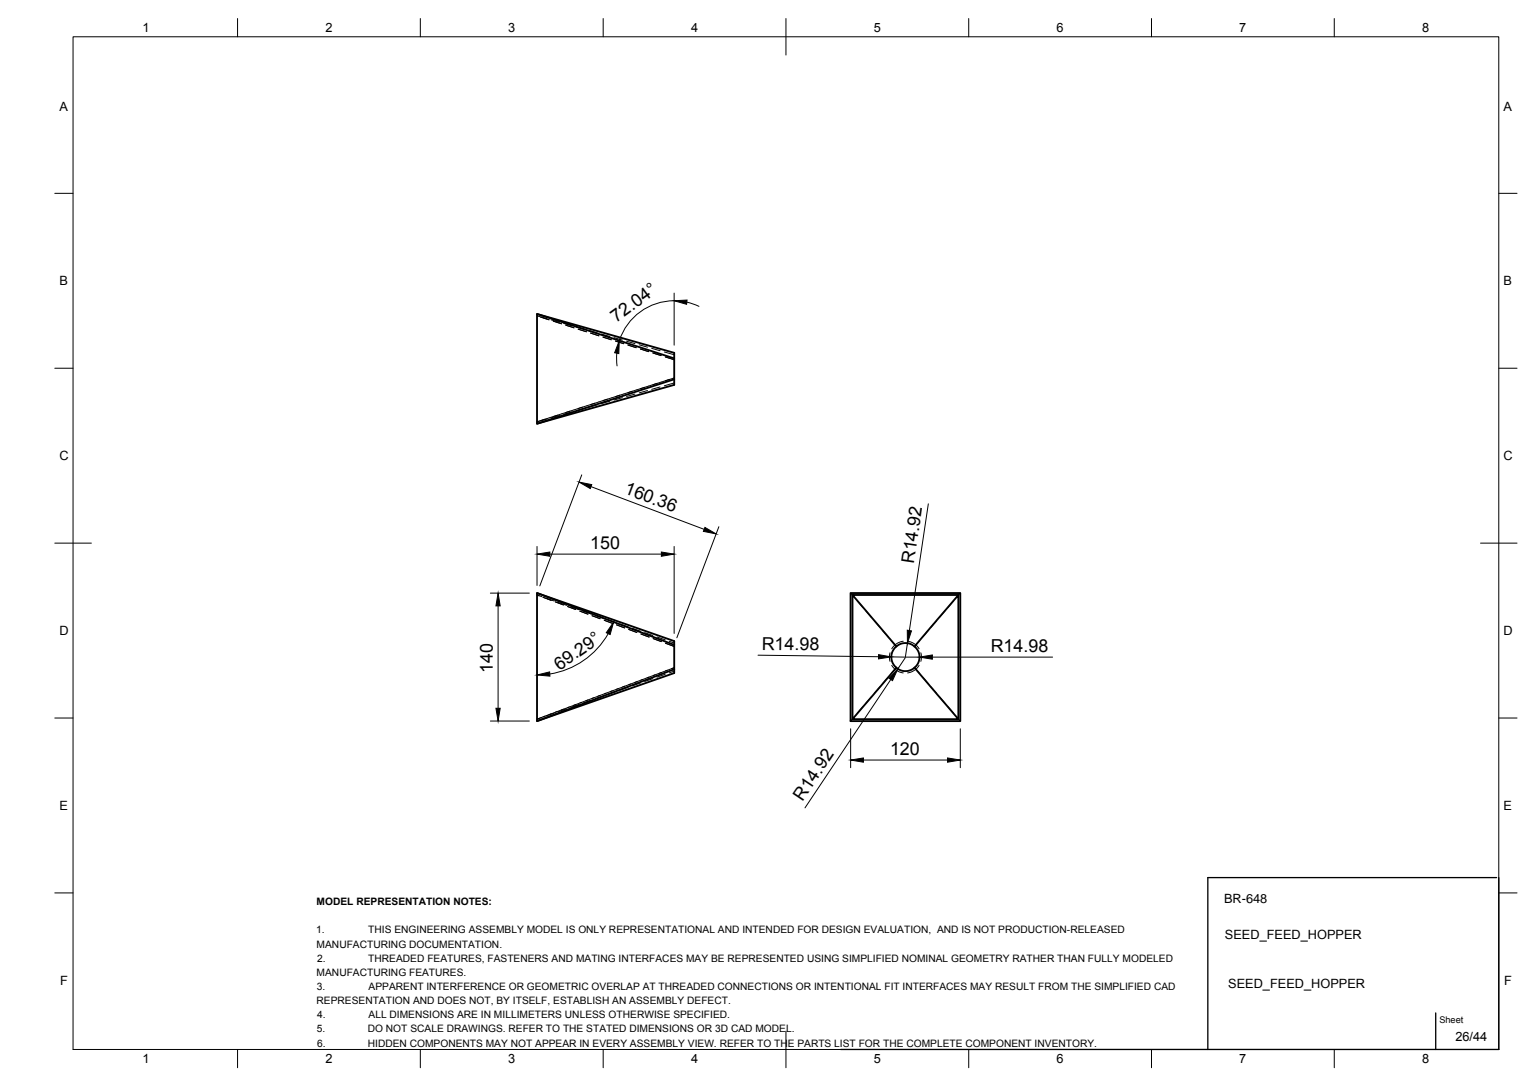
ISO-10303-21;
HEADER;
FILE_DESCRIPTION((''),'2;1');
FILE_NAME('SEED_FEED_HOPPER.step','2026-10-01T22:05:39-07:00',(''),(''),'','','');
FILE_SCHEMA (('AUTOMOTIVE_DESIGN { 1 0 10303 214 3 1 1 }'));
ENDSEC;
DATA;
#10=MECHANICAL_DESIGN_GEOMETRIC_PRESENTATION_REPRESENTATION('',(#624),#24628);
#13=B_SPLINE_SURFACE_WITH_KNOTS('',3,3,((#22362,#22363,#22364,#22365,#22366,
#22367,#22368),(#22369,#22370,#22371,#22372,#22373,#22374,#22375),(#22376,
#22377,#22378,#22379,#22380,#22381,#22382),(#22383,#22384,#22385,#22386,
#22387,#22388,#22389),(#22390,#22391,#22392,#22393,#22394,#22395,#22396),
(#22397,#22398,#22399,#22400,#22401,#22402,#22403)),.UNSPECIFIED.,.F.,.F.,
 .F.,(4,1,1,4),(4,1,1,1,4),(-0.0016506318429804,0.2850068720673,0.571664375977581,
1.001650631843),(0.00440207412461945,0.433637210821686,0.71979396861973,
0.862872347518753,1.00595072641777),.UNSPECIFIED.) ;
#14=B_SPLINE_SURFACE_WITH_KNOTS('',3,3,((#22475,#22476,#22477,#22478,#22479,
#22480,#22481),(#22482,#22483,#22484,#22485,#22486,#22487,#22488),(#22489,
#22490,#22491,#22492,#22493,#22494,#22495),(#22496,#22497,#22498,#22499,
#22500,#22501,#22502),(#22503,#22504,#22505,#22506,#22507,#22508,#22509),
(#22510,#22511,#22512,#22513,#22514,#22515,#22516),(#22517,#22518,#22519,
#22520,#22521,#22522,#22523)),.UNSPECIFIED.,.F.,.F.,.F.,(4,1,1,1,4),(4,
1,1,1,4),(-0.00135073644513769,0.285135398666339,0.428378466222077,0.714864601333554,
1.00135073644503),(0.00363062073752213,0.433196670488858,0.719574036989748,
0.862762720240194,1.00595140349064),.UNSPECIFIED.) ;
#15=B_SPLINE_SURFACE_WITH_KNOTS('',3,3,((#22568,#22569,#22570,#22571,#22572,
#22573),(#22574,#22575,#22576,#22577,#22578,#22579),(#22580,#22581,#22582,
#22583,#22584,#22585),(#22586,#22587,#22588,#22589,#22590,#22591),(#22592,
#22593,#22594,#22595,#22596,#22597),(#22598,#22599,#22600,#22601,#22602,
#22603)),.UNSPECIFIED.,.F.,.F.,.F.,(4,1,1,4),(4,1,1,4),(-0.00165063184293244,
0.28500687206736,0.571664375977652,1.00165063184309),(0.00440207412461947,
0.576715589720881,0.862872347519012,1.00595072641808),.UNSPECIFIED.) ;
#16=B_SPLINE_SURFACE_WITH_KNOTS('',3,3,((#22646,#22647,#22648,#22649,#22650,
#22651,#22652),(#22653,#22654,#22655,#22656,#22657,#22658,#22659),(#22660,
#22661,#22662,#22663,#22664,#22665,#22666),(#22667,#22668,#22669,#22670,
#22671,#22672,#22673),(#22674,#22675,#22676,#22677,#22678,#22679,#22680),
(#22681,#22682,#22683,#22684,#22685,#22686,#22687),(#22688,#22689,#22690,
#22691,#22692,#22693,#22694)),.UNSPECIFIED.,.F.,.F.,.F.,(4,1,1,1,4),(4,
1,1,1,4),(-0.00135073644515613,0.141892331110593,0.428378466222092,0.714864601333591,
1.00135073644509),(0.00363062073752213,0.433196670488988,0.719574036989965,
0.862762720240453,1.00595140349094),.UNSPECIFIED.) ;
#17=B_SPLINE_SURFACE_WITH_KNOTS('',3,3,((#22731,#22732,#22733,#22734),(#22735,
#22736,#22737,#22738),(#22739,#22740,#22741,#22742),(#22743,#22744,#22745,
#22746),(#22747,#22748,#22749,#22750),(#22751,#22752,#22753,#22754)),
 .UNSPECIFIED.,.F.,.F.,.F.,(4,1,1,4),(4,4),(0.,0.285714285714286,0.571428571428571,
1.),(0.,1.),.UNSPECIFIED.) ;
#18=B_SPLINE_SURFACE_WITH_KNOTS('',3,3,((#22757,#22758,#22759,#22760),(#22761,
#22762,#22763,#22764),(#22765,#22766,#22767,#22768),(#22769,#22770,#22771,
#22772),(#22773,#22774,#22775,#22776),(#22777,#22778,#22779,#22780),(#22781,
#22782,#22783,#22784)),.UNSPECIFIED.,.F.,.F.,.F.,(4,1,1,1,4),(4,4),(0.,
0.285714285714286,0.571428571428571,0.857142857142857,1.),(0.,1.),
 .UNSPECIFIED.) ;
#19=B_SPLINE_SURFACE_WITH_KNOTS('',3,3,((#22786,#22787,#22788,#22789),(#22790,
#22791,#22792,#22793),(#22794,#22795,#22796,#22797),(#22798,#22799,#22800,
#22801),(#22802,#22803,#22804,#22805),(#22806,#22807,#22808,#22809)),
 .UNSPECIFIED.,.F.,.F.,.F.,(4,1,1,4),(4,4),(0.,0.285714285714286,0.571428571428571,
1.),(0.,1.),.UNSPECIFIED.) ;
#20=B_SPLINE_SURFACE_WITH_KNOTS('',3,3,((#22811,#22812,#22813,#22814),(#22815,
#22816,#22817,#22818),(#22819,#22820,#22821,#22822),(#22823,#22824,#22825,
#22826),(#22827,#22828,#22829,#22830),(#22831,#22832,#22833,#22834),(#22835,
#22836,#22837,#22838)),.UNSPECIFIED.,.F.,.F.,.F.,(4,1,1,1,4),(4,4),(0.,
0.285714285714286,0.571428571428571,0.857142857142857,1.),(0.,1.),
 .UNSPECIFIED.) ;
#540=SHAPE_REPRESENTATION_RELATIONSHIP('SRR','None',#24813,#582) ;
#582=ADVANCED_BREP_SHAPE_REPRESENTATION('',(#663),#24603) ;
#624=STYLED_ITEM('',(#25038),#663) ;
#663=MANIFOLD_SOLID_BREP('SEED_FEED_HOPPER',#13166) ;
#871=FACE_BOUND('',#4402,.T.) ;
#872=FACE_BOUND('',#4404,.T.) ;
#964=B_SPLINE_CURVE_WITH_KNOTS('',3,(#22406,#22407,#22408,#22409,#22410,
#22411),.UNSPECIFIED.,.F.,.F.,(4,2,4),(0.306797486954004,6.07243999004955,
11.9854458646039),.UNSPECIFIED.) ;
#965=B_SPLINE_CURVE_WITH_KNOTS('',3,(#22413,#22414,#22415,#22416,#22417,
#22418,#22419,#22420,#22421,#22422,#22423,#22424,#22425,#22426,#22427,#22428),
 .UNSPECIFIED.,.F.,.F.,(4,3,3,3,3,4),(-22.7491660875703,-22.7326322777483,
-11.3663161388741,-8.43127796455208,-7.52321841795695,-0.0683548158626444),
 .UNSPECIFIED.) ;
#966=B_SPLINE_CURVE_WITH_KNOTS('',3,(#22430,#22431,#22432,#22433,#22434,
#22435,#22436),.UNSPECIFIED.,.F.,.F.,(4,3,4),(0.149401224909902,0.242876764795977,
0.248953560391612),.UNSPECIFIED.) ;
#967=B_SPLINE_CURVE_WITH_KNOTS('',3,(#22438,#22439,#22440,#22441,#22442,
#22443,#22444,#22445,#22446,#22447),.UNSPECIFIED.,.F.,.F.,(4,2,2,2,4),(0.0182113449411267,
0.579498375271715,1.16103870949885,1.68899220567266,2.20049000979166),
 .UNSPECIFIED.) ;
#968=B_SPLINE_CURVE_WITH_KNOTS('',3,(#22449,#22450,#22451,#22452,#22453,
#22454,#22455),.UNSPECIFIED.,.F.,.F.,(4,3,4),(-0.00607546474194351,0.,0.0934550397936403),
 .UNSPECIFIED.) ;
#969=B_SPLINE_CURVE_WITH_KNOTS('',3,(#22456,#22457,#22458,#22459,#22460,
#22461,#22462,#22463,#22464,#22465,#22466,#22467,#22468,#22469,#22470,#22471,
#22472,#22473,#22474),.UNSPECIFIED.,.F.,.F.,(4,3,3,3,3,3,4),(-8.32916619482315,
-6.19701983076071,-5.68275153370131,-5.33626613109357,-0.491091685615563,
0.,0.00607621245833095),.UNSPECIFIED.) ;
#970=B_SPLINE_CURVE_WITH_KNOTS('',3,(#22525,#22526,#22527,#22528,#22529,
#22530),.UNSPECIFIED.,.F.,.F.,(4,2,4),(0.330130434724689,7.1450073655251,
14.1316592404919),.UNSPECIFIED.) ;
#971=B_SPLINE_CURVE_WITH_KNOTS('',3,(#22532,#22533,#22534,#22535,#22536,
#22537,#22538,#22539,#22540,#22541,#22542,#22543,#22544,#22545,#22546,#22547),
 .UNSPECIFIED.,.F.,.F.,(4,3,3,3,3,4),(-0.00607619681590831,0.,4.17713740634383,
5.25576768694509,5.58948106622994,8.32915431888067),.UNSPECIFIED.) ;
#972=B_SPLINE_CURVE_WITH_KNOTS('',3,(#22549,#22550,#22551,#22552,#22553,
#22554,#22555),.UNSPECIFIED.,.F.,.F.,(4,3,4),(-0.093455064791989,0.,0.00607547210165982),
 .UNSPECIFIED.) ;
#973=B_SPLINE_CURVE_WITH_KNOTS('',3,(#22556,#22557,#22558,#22559,#22560,
#22561,#22562,#22563,#22564,#22565,#22566,#22567),.UNSPECIFIED.,.F.,.F.,
(4,2,2,2,2,4),(0.0230676064321383,0.582322749083777,1.16480388155931,1.75243736265584,
2.22755255780229,2.68204291945575),.UNSPECIFIED.) ;
#974=B_SPLINE_CURVE_WITH_KNOTS('',3,(#22605,#22606,#22607,#22608,#22609,
#22610),.UNSPECIFIED.,.F.,.F.,(4,2,4),(0.306797486954258,6.07243999011767,
11.9854458647428),.UNSPECIFIED.) ;
#975=B_SPLINE_CURVE_WITH_KNOTS('',3,(#22612,#22613,#22614,#22615,#22616,
#22617,#22618,#22619,#22620,#22621,#22622,#22623,#22624,#22625,#22626,#22627),
 .UNSPECIFIED.,.F.,.F.,(4,3,3,3,3,4),(-22.7491696598115,-22.732635833168,
-11.366317916584,-8.43127594084112,-7.52321777514952,-0.0683548158626444),
 .UNSPECIFIED.) ;
#976=B_SPLINE_CURVE_WITH_KNOTS('',3,(#22629,#22630,#22631,#22632,#22633,
#22634,#22635),.UNSPECIFIED.,.F.,.F.,(4,3,4),(0.149401210175699,0.242876791624169,
0.248953579588731),.UNSPECIFIED.) ;
#977=B_SPLINE_CURVE_WITH_KNOTS('',3,(#22636,#22637,#22638,#22639,#22640,
#22641,#22642,#22643,#22644,#22645),.UNSPECIFIED.,.F.,.F.,(4,2,2,2,4),(0.0182113449411156,
0.579498375271719,1.16103870949884,1.68899220567264,2.20049000979168),
 .UNSPECIFIED.) ;
#978=B_SPLINE_CURVE_WITH_KNOTS('',3,(#22695,#22696,#22697,#22698,#22699,
#22700),.UNSPECIFIED.,.F.,.F.,(4,2,4),(0.330130434724726,7.14500736553715,
14.1316592405166),.UNSPECIFIED.) ;
#979=B_SPLINE_CURVE_WITH_KNOTS('',3,(#22701,#22702,#22703,#22704,#22705,
#22706,#22707,#22708,#22709,#22710,#22711,#22712),.UNSPECIFIED.,.F.,.F.,
(4,2,2,2,2,4),(0.0230676064320783,0.582322749083774,1.1648038815593,1.75243736265581,
2.22755255780225,2.68204291945565),.UNSPECIFIED.) ;
#1442=LINE('',#22725,#2278) ;
#1443=LINE('',#22727,#2279) ;
#1444=LINE('',#22729,#2280) ;
#1445=LINE('',#22730,#2281) ;
#1446=LINE('',#22755,#2282) ;
#1447=LINE('',#22756,#2283) ;
#1448=LINE('',#22785,#2284) ;
#1449=LINE('',#22810,#2285) ;
#2278=VECTOR('',#18253,1.) ;
#2279=VECTOR('',#18254,1.) ;
#2280=VECTOR('',#18255,1.) ;
#2281=VECTOR('',#18256,1.) ;
#2282=VECTOR('',#18257,16.7569118395806) ;
#2283=VECTOR('',#18258,16.7569118395806) ;
#2284=VECTOR('',#18259,16.7569118395806) ;
#2285=VECTOR('',#18260,16.7569118395806) ;
#3445=FACE_OUTER_BOUND('',#4397,.T.) ;
#3446=FACE_OUTER_BOUND('',#4398,.T.) ;
#3447=FACE_OUTER_BOUND('',#4399,.T.) ;
#3448=FACE_OUTER_BOUND('',#4400,.T.) ;
#3449=FACE_OUTER_BOUND('',#4401,.T.) ;
#3450=FACE_OUTER_BOUND('',#4403,.T.) ;
#3451=FACE_OUTER_BOUND('',#4405,.T.) ;
#3452=FACE_OUTER_BOUND('',#4406,.T.) ;
#3453=FACE_OUTER_BOUND('',#4407,.T.) ;
#3454=FACE_OUTER_BOUND('',#4408,.T.) ;
#4397=EDGE_LOOP('',(#10729,#10730,#10731,#10732,#10733,#10734)) ;
#4398=EDGE_LOOP('',(#10735,#10736,#10737,#10738,#10739,#10740)) ;
#4399=EDGE_LOOP('',(#10741,#10742,#10743,#10744,#10745,#10746)) ;
#4400=EDGE_LOOP('',(#10747,#10748,#10749,#10750,#10751,#10752)) ;
#4401=EDGE_LOOP('',(#10753,#10754,#10755,#10756)) ;
#4402=EDGE_LOOP('',(#10757,#10758,#10759,#10760)) ;
#4403=EDGE_LOOP('',(#10761,#10762,#10763,#10764)) ;
#4404=EDGE_LOOP('',(#10765,#10766,#10767,#10768)) ;
#4405=EDGE_LOOP('',(#10769,#10770,#10771,#10772)) ;
#4406=EDGE_LOOP('',(#10773,#10774,#10775,#10776)) ;
#4407=EDGE_LOOP('',(#10777,#10778,#10779,#10780)) ;
#4408=EDGE_LOOP('',(#10781,#10782,#10783,#10784)) ;
#5342=CIRCLE('',#14858,1.75) ;
#5343=CIRCLE('',#14859,1.75) ;
#5344=CIRCLE('',#14860,1.75) ;
#5345=CIRCLE('',#14861,1.75) ;
#6312=VERTEX_POINT('',#22404) ;
#6313=VERTEX_POINT('',#22405) ;
#6314=VERTEX_POINT('',#22412) ;
#6315=VERTEX_POINT('',#22429) ;
#6316=VERTEX_POINT('',#22437) ;
#6317=VERTEX_POINT('',#22448) ;
#6318=VERTEX_POINT('',#22524) ;
#6319=VERTEX_POINT('',#22531) ;
#6320=VERTEX_POINT('',#22548) ;
#6321=VERTEX_POINT('',#22604) ;
#6322=VERTEX_POINT('',#22611) ;
#6323=VERTEX_POINT('',#22628) ;
#6324=VERTEX_POINT('',#22714) ;
#6325=VERTEX_POINT('',#22715) ;
#6326=VERTEX_POINT('',#22717) ;
#6327=VERTEX_POINT('',#22719) ;
#6328=VERTEX_POINT('',#22723) ;
#6329=VERTEX_POINT('',#22724) ;
#6330=VERTEX_POINT('',#22726) ;
#6331=VERTEX_POINT('',#22728) ;
#7854=EDGE_CURVE('',#6312,#6313,#964,.T.) ;
#7855=EDGE_CURVE('',#6312,#6314,#965,.F.) ;
#7856=EDGE_CURVE('',#6314,#6315,#966,.F.) ;
#7857=EDGE_CURVE('',#6316,#6315,#967,.T.) ;
#7858=EDGE_CURVE('',#6317,#6316,#968,.T.) ;
#7859=EDGE_CURVE('',#6313,#6317,#969,.T.) ;
#7860=EDGE_CURVE('',#6318,#6312,#970,.T.) ;
#7861=EDGE_CURVE('',#6318,#6319,#971,.F.) ;
#7862=EDGE_CURVE('',#6319,#6320,#972,.F.) ;
#7863=EDGE_CURVE('',#6315,#6320,#973,.T.) ;
#7864=EDGE_CURVE('',#6321,#6318,#974,.T.) ;
#7865=EDGE_CURVE('',#6321,#6322,#975,.F.) ;
#7866=EDGE_CURVE('',#6322,#6323,#976,.F.) ;
#7867=EDGE_CURVE('',#6320,#6323,#977,.T.) ;
#7868=EDGE_CURVE('',#6313,#6321,#978,.T.) ;
#7869=EDGE_CURVE('',#6323,#6316,#979,.T.) ;
#7870=EDGE_CURVE('',#6324,#6325,#5342,.T.) ;
#7871=EDGE_CURVE('',#6326,#6324,#5343,.T.) ;
#7872=EDGE_CURVE('',#6327,#6326,#5344,.T.) ;
#7873=EDGE_CURVE('',#6325,#6327,#5345,.T.) ;
#7874=EDGE_CURVE('',#6328,#6329,#1442,.T.) ;
#7875=EDGE_CURVE('',#6329,#6330,#1443,.T.) ;
#7876=EDGE_CURVE('',#6330,#6331,#1444,.T.) ;
#7877=EDGE_CURVE('',#6331,#6328,#1445,.T.) ;
#7878=EDGE_CURVE('',#6328,#6324,#1446,.T.) ;
#7879=EDGE_CURVE('',#6329,#6325,#1447,.T.) ;
#7880=EDGE_CURVE('',#6330,#6327,#1448,.T.) ;
#7881=EDGE_CURVE('',#6331,#6326,#1449,.T.) ;
#10729=ORIENTED_EDGE('',*,*,#7854,.F.) ;
#10730=ORIENTED_EDGE('',*,*,#7855,.T.) ;
#10731=ORIENTED_EDGE('',*,*,#7856,.T.) ;
#10732=ORIENTED_EDGE('',*,*,#7857,.F.) ;
#10733=ORIENTED_EDGE('',*,*,#7858,.F.) ;
#10734=ORIENTED_EDGE('',*,*,#7859,.F.) ;
#10735=ORIENTED_EDGE('',*,*,#7860,.F.) ;
#10736=ORIENTED_EDGE('',*,*,#7861,.T.) ;
#10737=ORIENTED_EDGE('',*,*,#7862,.T.) ;
#10738=ORIENTED_EDGE('',*,*,#7863,.F.) ;
#10739=ORIENTED_EDGE('',*,*,#7856,.F.) ;
#10740=ORIENTED_EDGE('',*,*,#7855,.F.) ;
#10741=ORIENTED_EDGE('',*,*,#7864,.F.) ;
#10742=ORIENTED_EDGE('',*,*,#7865,.T.) ;
#10743=ORIENTED_EDGE('',*,*,#7866,.T.) ;
#10744=ORIENTED_EDGE('',*,*,#7867,.F.) ;
#10745=ORIENTED_EDGE('',*,*,#7862,.F.) ;
#10746=ORIENTED_EDGE('',*,*,#7861,.F.) ;
#10747=ORIENTED_EDGE('',*,*,#7868,.F.) ;
#10748=ORIENTED_EDGE('',*,*,#7859,.T.) ;
#10749=ORIENTED_EDGE('',*,*,#7858,.T.) ;
#10750=ORIENTED_EDGE('',*,*,#7869,.F.) ;
#10751=ORIENTED_EDGE('',*,*,#7866,.F.) ;
#10752=ORIENTED_EDGE('',*,*,#7865,.F.) ;
#10753=ORIENTED_EDGE('',*,*,#7870,.F.) ;
#10754=ORIENTED_EDGE('',*,*,#7871,.F.) ;
#10755=ORIENTED_EDGE('',*,*,#7872,.F.) ;
#10756=ORIENTED_EDGE('',*,*,#7873,.F.) ;
#10757=ORIENTED_EDGE('',*,*,#7857,.T.) ;
#10758=ORIENTED_EDGE('',*,*,#7863,.T.) ;
#10759=ORIENTED_EDGE('',*,*,#7867,.T.) ;
#10760=ORIENTED_EDGE('',*,*,#7869,.T.) ;
#10761=ORIENTED_EDGE('',*,*,#7874,.T.) ;
#10762=ORIENTED_EDGE('',*,*,#7875,.T.) ;
#10763=ORIENTED_EDGE('',*,*,#7876,.T.) ;
#10764=ORIENTED_EDGE('',*,*,#7877,.T.) ;
#10765=ORIENTED_EDGE('',*,*,#7854,.T.) ;
#10766=ORIENTED_EDGE('',*,*,#7868,.T.) ;
#10767=ORIENTED_EDGE('',*,*,#7864,.T.) ;
#10768=ORIENTED_EDGE('',*,*,#7860,.T.) ;
#10769=ORIENTED_EDGE('',*,*,#7874,.F.) ;
#10770=ORIENTED_EDGE('',*,*,#7878,.T.) ;
#10771=ORIENTED_EDGE('',*,*,#7870,.T.) ;
#10772=ORIENTED_EDGE('',*,*,#7879,.F.) ;
#10773=ORIENTED_EDGE('',*,*,#7875,.F.) ;
#10774=ORIENTED_EDGE('',*,*,#7879,.T.) ;
#10775=ORIENTED_EDGE('',*,*,#7873,.T.) ;
#10776=ORIENTED_EDGE('',*,*,#7880,.F.) ;
#10777=ORIENTED_EDGE('',*,*,#7876,.F.) ;
#10778=ORIENTED_EDGE('',*,*,#7880,.T.) ;
#10779=ORIENTED_EDGE('',*,*,#7872,.T.) ;
#10780=ORIENTED_EDGE('',*,*,#7881,.F.) ;
#10781=ORIENTED_EDGE('',*,*,#7877,.F.) ;
#10782=ORIENTED_EDGE('',*,*,#7881,.T.) ;
#10783=ORIENTED_EDGE('',*,*,#7871,.T.) ;
#10784=ORIENTED_EDGE('',*,*,#7878,.F.) ;
#12164=PLANE('',#14857) ;
#12165=PLANE('',#14862) ;
#12840=ADVANCED_FACE('',(#3445),#13,.T.) ;
#12841=ADVANCED_FACE('',(#3446),#14,.T.) ;
#12842=ADVANCED_FACE('',(#3447),#15,.T.) ;
#12843=ADVANCED_FACE('',(#3448),#16,.T.) ;
#12844=ADVANCED_FACE('',(#3449,#871),#12164,.F.) ;
#12845=ADVANCED_FACE('',(#3450,#872),#12165,.T.) ;
#12846=ADVANCED_FACE('',(#3451),#17,.F.) ;
#12847=ADVANCED_FACE('',(#3452),#18,.F.) ;
#12848=ADVANCED_FACE('',(#3453),#19,.F.) ;
#12849=ADVANCED_FACE('',(#3454),#20,.F.) ;
#13166=CLOSED_SHELL('',(#12840,#12841,#12842,#12843,#12844,#12845,#12846,
#12847,#12848,#12849)) ;
#14856=AXIS2_PLACEMENT_3D('',#22361,#18239,#18240) ;
#14857=AXIS2_PLACEMENT_3D('',#22713,#18241,#18242) ;
#14858=AXIS2_PLACEMENT_3D('',#22716,#18243,#18244) ;
#14859=AXIS2_PLACEMENT_3D('',#22718,#18245,#18246) ;
#14860=AXIS2_PLACEMENT_3D('',#22720,#18247,#18248) ;
#14861=AXIS2_PLACEMENT_3D('',#22721,#18249,#18250) ;
#14862=AXIS2_PLACEMENT_3D('',#22722,#18251,#18252) ;
#18239=DIRECTION('axis',(0.,0.,1.)) ;
#18240=DIRECTION('refdir',(1.,0.,0.)) ;
#18241=DIRECTION('center_axis',(0.,0.,1.)) ;
#18242=DIRECTION('ref_axis',(1.,0.,0.)) ;
#18243=DIRECTION('center_axis',(0.,0.,1.)) ;
#18244=DIRECTION('ref_axis',(1.,0.,0.)) ;
#18245=DIRECTION('center_axis',(0.,0.,1.)) ;
#18246=DIRECTION('ref_axis',(1.,0.,0.)) ;
#18247=DIRECTION('center_axis',(0.,0.,1.)) ;
#18248=DIRECTION('ref_axis',(1.,0.,0.)) ;
#18249=DIRECTION('center_axis',(0.,0.,1.)) ;
#18250=DIRECTION('ref_axis',(1.,0.,0.)) ;
#18251=DIRECTION('center_axis',(0.,0.,1.)) ;
#18252=DIRECTION('ref_axis',(1.,0.,0.)) ;
#18253=DIRECTION('',(0.,-1.,0.)) ;
#18254=DIRECTION('',(1.,0.,0.)) ;
#18255=DIRECTION('',(0.,1.,0.)) ;
#18256=DIRECTION('',(-1.,-6.34413156928661E-17,0.)) ;
#18257=DIRECTION('',(0.338445472540165,-0.290096119320142,-0.895153005732796)) ;
#18258=DIRECTION('',(0.338445472540165,0.290096119320142,-0.895153005732796)) ;
#18259=DIRECTION('',(-0.338445472540165,0.290096119320142,-0.895153005732796)) ;
#18260=DIRECTION('',(-0.338445472540165,-0.290096119320142,-0.895153005732796)) ;
#22361=CARTESIAN_POINT('',(0.,0.,0.)) ;
#22362=CARTESIAN_POINT('Ctrl Pts',(-29.7879704997762,4.1982235964065,15.004760387006)) ;
#22363=CARTESIAN_POINT('Ctrl Pts',(-28.9765416158345,3.49667700708559,12.8596184051575)) ;
#22364=CARTESIAN_POINT('Ctrl Pts',(-27.6245525523466,2.32566824542574,9.28480711044218)) ;
#22365=CARTESIAN_POINT('Ctrl Pts',(-26.005233549839,0.90734538201738,4.99813706529367)) ;
#22366=CARTESIAN_POINT('Ctrl Pts',(-24.9352460971343,-0.0565633455803164,
2.14271187262585)) ;
#22367=CARTESIAN_POINT('Ctrl Pts',(-24.4110437339872,-0.552959968693851,
0.715613732723115)) ;
#22368=CARTESIAN_POINT('Ctrl Pts',(-24.1589049321087,-0.806397566452131,
-5.70268832156273E-10)) ;
#22369=CARTESIAN_POINT('Ctrl Pts',(-29.7880085856475,3.05586778828661,15.0030622151785)) ;
#22370=CARTESIAN_POINT('Ctrl Pts',(-28.9985961339778,2.49325092521034,12.8575620409374)) ;
#22371=CARTESIAN_POINT('Ctrl Pts',(-27.6830843893262,1.55403581881225,9.28200460526821)) ;
#22372=CARTESIAN_POINT('Ctrl Pts',(-26.1062403134519,0.416417293310764,
4.99328651815293)) ;
#22373=CARTESIAN_POINT('Ctrl Pts',(-25.0612351613324,-0.357449889914694,
2.13576141937932)) ;
#22374=CARTESIAN_POINT('Ctrl Pts',(-24.5450981755029,-0.75720095086868,
0.707828841054705)) ;
#22375=CARTESIAN_POINT('Ctrl Pts',(-24.2953334946171,-0.964113147540073,
-0.00706604193771441)) ;
#22376=CARTESIAN_POINT('Ctrl Pts',(-29.7880984019284,0.77088432617787,15.0004371510981)) ;
#22377=CARTESIAN_POINT('Ctrl Pts',(-29.0320656779143,0.477248554069186,
12.854352481685)) ;
#22378=CARTESIAN_POINT('Ctrl Pts',(-27.7718140786327,-0.0129653268429286,
9.2776079223855)) ;
#22379=CARTESIAN_POINT('Ctrl Pts',(-26.2598801085757,-0.606556867865899,
4.9857552974963)) ;
#22380=CARTESIAN_POINT('Ctrl Pts',(-25.252746996273,-1.01128931246026,2.12475519883151)) ;
#22381=CARTESIAN_POINT('Ctrl Pts',(-24.7498599068977,-1.22062620685322,
0.694492730733407)) ;
#22382=CARTESIAN_POINT('Ctrl Pts',(-24.5000082407848,-1.33280874531094,
-0.0206610680077742)) ;
#22383=CARTESIAN_POINT('Ctrl Pts',(-29.7881434031396,-3.22828201380981,
14.9994444092913)) ;
#22384=CARTESIAN_POINT('Ctrl Pts',(-29.0444129979685,-3.06557811875762,
12.8531317839584)) ;
#22385=CARTESIAN_POINT('Ctrl Pts',(-27.8048257006081,-2.79391277080305,
9.27588292843548)) ;
#22386=CARTESIAN_POINT('Ctrl Pts',(-26.317044506741,-2.46505212911362,4.98280140110366)) ;
#22387=CARTESIAN_POINT('Ctrl Pts',(-25.3239448603091,-2.24067401478496,
2.12040334815057)) ;
#22388=CARTESIAN_POINT('Ctrl Pts',(-24.8262703953289,-2.12469662243215,
0.688894444476874)) ;
#22389=CARTESIAN_POINT('Ctrl Pts',(-24.5752760211477,-2.06194576114233,
-0.0267624859759424)) ;
#22390=CARTESIAN_POINT('Ctrl Pts',(-29.7880276285832,-6.08468988422692,
15.0022131292648)) ;
#22391=CARTESIAN_POINT('Ctrl Pts',(-29.0097274305354,-5.59160872404636,
12.8565299181811)) ;
#22392=CARTESIAN_POINT('Ctrl Pts',(-27.7122818351144,-4.76817410676846,
9.28063964648335)) ;
#22393=CARTESIAN_POINT('Ctrl Pts',(-26.1568276984181,-3.77112949936236,
4.99094264430357)) ;
#22394=CARTESIAN_POINT('Ctrl Pts',(-25.1243483646472,-3.09226178271257,
2.13236773367943)) ;
#22395=CARTESIAN_POINT('Ctrl Pts',(-24.6123236175051,-2.74112531762835,
0.704011231405586)) ;
#22396=CARTESIAN_POINT('Ctrl Pts',(-24.3635477758713,-2.557029061916,-0.0105990626214356)) ;
#22397=CARTESIAN_POINT('Ctrl Pts',(-29.7879704997762,-7.79822359640676,
15.004760387006)) ;
#22398=CARTESIAN_POINT('Ctrl Pts',(-28.9765416158345,-7.09667700708582,
12.8596184051575)) ;
#22399=CARTESIAN_POINT('Ctrl Pts',(-27.6245525523466,-5.92566824542591,
9.28480711044218)) ;
#22400=CARTESIAN_POINT('Ctrl Pts',(-26.0052335498389,-4.50734538201749,
4.99813706529367)) ;
#22401=CARTESIAN_POINT('Ctrl Pts',(-24.9352460971343,-3.54343665441975,
2.14271187262586)) ;
#22402=CARTESIAN_POINT('Ctrl Pts',(-24.4110437339872,-3.0470400313062,0.715613732723117)) ;
#22403=CARTESIAN_POINT('Ctrl Pts',(-24.1589049321087,-2.79360243354791,
-5.70267222332888E-10)) ;
#22404=CARTESIAN_POINT('',(-29.7862997944388,-7.58988663107372,15.)) ;
#22405=CARTESIAN_POINT('',(-29.7862997944388,3.98988663107372,15.)) ;
#22406=CARTESIAN_POINT('Ctrl Pts',(-29.7862997944388,-7.58988663107372,
15.)) ;
#22407=CARTESIAN_POINT('Ctrl Pts',(-29.7874854452745,-5.67140621570733,
15.)) ;
#22408=CARTESIAN_POINT('Ctrl Pts',(-29.7880884026998,-3.78346330304678,
15.)) ;
#22409=CARTESIAN_POINT('Ctrl Pts',(-29.7881190038692,0.0862220953979725,
15.)) ;
#22410=CARTESIAN_POINT('Ctrl Pts',(-29.7875160987196,2.02180642423597,15.)) ;
#22411=CARTESIAN_POINT('Ctrl Pts',(-29.7862997944388,3.98988663107372,15.)) ;
#22412=CARTESIAN_POINT('',(-24.1927688881933,-2.82237333273713,0.0891518022986763)) ;
#22413=CARTESIAN_POINT('Ctrl Pts',(-24.1927688881933,-2.82237333273713,
0.0891518022986763)) ;
#22414=CARTESIAN_POINT('Ctrl Pts',(-24.1934570101164,-2.82295781734209,
0.0909648418835227)) ;
#22415=CARTESIAN_POINT('Ctrl Pts',(-24.1941451106354,-2.82354227530196,
0.092777911525871)) ;
#22416=CARTESIAN_POINT('Ctrl Pts',(-24.1948331817638,-2.82412669991032,
0.094590989728832)) ;
#22417=CARTESIAN_POINT('Ctrl Pts',(-24.6678538621346,-3.22589464870741,
1.34100789310195)) ;
#22418=CARTESIAN_POINT('Ctrl Pts',(-25.0587313958119,-3.55537106707809,
2.39676629444992)) ;
#22419=CARTESIAN_POINT('Ctrl Pts',(-26.0013963074572,-4.35779250443395,
4.91745743939535)) ;
#22420=CARTESIAN_POINT('Ctrl Pts',(-26.2448135648579,-4.56499574616668,
5.56835652100608)) ;
#22421=CARTESIAN_POINT('Ctrl Pts',(-26.5249696032859,-4.803694805458,6.31696827513027)) ;
#22422=CARTESIAN_POINT('Ctrl Pts',(-26.852785444491,-5.0833030095669,7.19178833495937)) ;
#22423=CARTESIAN_POINT('Ctrl Pts',(-26.9542070569034,-5.16980985682658,
7.46244536212537)) ;
#22424=CARTESIAN_POINT('Ctrl Pts',(-27.0601952624917,-5.26023714996938,
7.74519169930263)) ;
#22425=CARTESIAN_POINT('Ctrl Pts',(-27.1656849213349,-5.35026234294172,
8.02651094121919)) ;
#22426=CARTESIAN_POINT('Ctrl Pts',(-28.0317195564602,-6.0893389121793,10.3360473422142)) ;
#22427=CARTESIAN_POINT('Ctrl Pts',(-28.9467094713777,-6.87166395755108,
12.769529848754)) ;
#22428=CARTESIAN_POINT('Ctrl Pts',(-29.7862997944388,-7.58988663107372,
15.)) ;
#22429=CARTESIAN_POINT('',(-24.1589049319639,-2.79360243342489,-4.75519821435677E-10)) ;
#22430=CARTESIAN_POINT('Ctrl Pts',(-24.1589049321088,-2.79360243354777,
-5.70273040595426E-10)) ;
#22431=CARTESIAN_POINT('Ctrl Pts',(-24.1695174648536,-2.80262121435912,
0.0279159200689838)) ;
#22432=CARTESIAN_POINT('Ctrl Pts',(-24.1801188171535,-2.81162839675808,
0.0558294517448662)) ;
#22433=CARTESIAN_POINT('Ctrl Pts',(-24.1907006565412,-2.82061729735981,
0.083715933657329)) ;
#22434=CARTESIAN_POINT('Ctrl Pts',(-24.1913885763442,-2.82120166105167,
0.0855288191530417)) ;
#22435=CARTESIAN_POINT('Ctrl Pts',(-24.1920764667909,-2.82178599256751,
0.0873417302858431)) ;
#22436=CARTESIAN_POINT('Ctrl Pts',(-24.1927643256631,-2.8223702901168,0.0891546605139208)) ;
#22437=CARTESIAN_POINT('',(-24.1589049319644,-0.806397566574673,-4.7482698675716E-10)) ;
#22438=CARTESIAN_POINT('Ctrl Pts',(-24.1589049323255,-0.8063975662679,1.09620886621735E-16)) ;
#22439=CARTESIAN_POINT('Ctrl Pts',(-24.283597624207,-0.945716532508702,
1.09623628239148E-16)) ;
#22440=CARTESIAN_POINT('Ctrl Pts',(-24.3808054594196,-1.10713716355173,
-1.18390020009684E-12)) ;
#22441=CARTESIAN_POINT('Ctrl Pts',(-24.512802414918,-1.46434976621459,-1.18390020009684E-12)) ;
#22442=CARTESIAN_POINT('Ctrl Pts',(-24.5438655539448,-1.6575893537085,-1.38777878078145E-15)) ;
#22443=CARTESIAN_POINT('Ctrl Pts',(-24.5311976151215,-2.02703780425878,
-1.38777878078145E-15)) ;
#22444=CARTESIAN_POINT('Ctrl Pts',(-24.4941869311108,-2.20048822446343,
1.4585554986013E-14)) ;
#22445=CARTESIAN_POINT('Ctrl Pts',(-24.3634307218009,-2.52123101046768,
1.4585554986013E-14)) ;
#22446=CARTESIAN_POINT('Ctrl Pts',(-24.2725344551939,-2.66664433040153,
3.20484281317344E-16)) ;
#22447=CARTESIAN_POINT('Ctrl Pts',(-24.1589049323255,-2.79360243373209,
3.20484666411866E-16)) ;
#22448=CARTESIAN_POINT('',(-24.1927688881933,-0.777626667262871,0.0891518022986696)) ;
#22449=CARTESIAN_POINT('Ctrl Pts',(-24.1927640983708,-0.777630284368101,
0.0891545456106432)) ;
#22450=CARTESIAN_POINT('Ctrl Pts',(-24.1920762479986,-0.778214559997417,
0.0873416191464197)) ;
#22451=CARTESIAN_POINT('Ctrl Pts',(-24.1913883666309,-0.778798869477654,
0.0855287137798584)) ;
#22452=CARTESIAN_POINT('Ctrl Pts',(-24.1907004548719,-0.779383212398548,
0.0837158318083245)) ;
#22453=CARTESIAN_POINT('Ctrl Pts',(-24.1801187424362,-0.788371790761656,
0.0558294125816257)) ;
#22454=CARTESIAN_POINT('Ctrl Pts',(-24.1695174641247,-0.797378786260146,
0.0279159181518874)) ;
#22455=CARTESIAN_POINT('Ctrl Pts',(-24.158904932109,-0.806397566451893,
-5.69441659411157E-10)) ;
#22456=CARTESIAN_POINT('Ctrl Pts',(-29.7862997944388,3.98988663107372,15.)) ;
#22457=CARTESIAN_POINT('Ctrl Pts',(-29.1328907328544,3.43093163811475,13.2641422031832)) ;
#22458=CARTESIAN_POINT('Ctrl Pts',(-28.4338012516642,2.8331537658536,11.4053304313931)) ;
#22459=CARTESIAN_POINT('Ctrl Pts',(-27.7476813820024,2.24714826965254,9.5776689963089)) ;
#22460=CARTESIAN_POINT('Ctrl Pts',(-27.5821910090633,2.10580522975702,9.13684169211246)) ;
#22461=CARTESIAN_POINT('Ctrl Pts',(-27.4174547163538,1.96514782273,8.69782652065271)) ;
#22462=CARTESIAN_POINT('Ctrl Pts',(-27.2542924969021,1.82588555176052,8.26278713091792)) ;
#22463=CARTESIAN_POINT('Ctrl Pts',(-27.144362859745,1.73205837186077,7.96968176361375)) ;
#22464=CARTESIAN_POINT('Ctrl Pts',(-27.0345809892665,1.63838104542639,7.67686898630538)) ;
#22465=CARTESIAN_POINT('Ctrl Pts',(-26.926973332117,1.54658537416295,7.38975189096568)) ;
#22466=CARTESIAN_POINT('Ctrl Pts',(-25.4222119002236,0.262935219600215,
3.37477058806011)) ;
#22467=CARTESIAN_POINT('Ctrl Pts',(-24.8950276354157,-0.182007944164745,
1.94978881746105)) ;
#22468=CARTESIAN_POINT('Ctrl Pts',(-24.3591765397677,-0.636412221527215,
0.52907137988932)) ;
#22469=CARTESIAN_POINT('Ctrl Pts',(-24.304864353331,-0.682469213908392,
0.385071916288646)) ;
#22470=CARTESIAN_POINT('Ctrl Pts',(-24.2504445757749,-0.728638841618619,
0.241127884134561)) ;
#22471=CARTESIAN_POINT('Ctrl Pts',(-24.1948331817649,-0.775873300087209,
0.0945909897337519)) ;
#22472=CARTESIAN_POINT('Ctrl Pts',(-24.1941451093438,-0.776457725793072,
0.0927779081250757)) ;
#22473=CARTESIAN_POINT('Ctrl Pts',(-24.1934570114089,-0.777042181560007,
0.0909648452891593)) ;
#22474=CARTESIAN_POINT('Ctrl Pts',(-24.1927688881933,-0.777626667262871,
0.0891518022986696)) ;
#22475=CARTESIAN_POINT('Ctrl Pts',(-29.9981473192967,-7.59210557221634,
15.0072731137197)) ;
#22476=CARTESIAN_POINT('Ctrl Pts',(-29.1792583701285,-6.89610811582497,
12.86098396712)) ;
#22477=CARTESIAN_POINT('Ctrl Pts',(-27.8122956599382,-5.73660744609276,
9.28448922209497)) ;
#22478=CARTESIAN_POINT('Ctrl Pts',(-26.155155413787,-4.35020365083683,4.99743947373446)) ;
#22479=CARTESIAN_POINT('Ctrl Pts',(-25.0283996405944,-3.44029824352441,
2.14308849921247)) ;
#22480=CARTESIAN_POINT('Ctrl Pts',(-24.4500092405164,-3.00195022998226,
0.716220735767208)) ;
#22481=CARTESIAN_POINT('Ctrl Pts',(-24.1589049321088,-2.79360243354776,
-5.70272704059072E-10)) ;
#22482=CARTESIAN_POINT('Ctrl Pts',(-28.6654023870952,-7.59208088863895,
15.0047443273315)) ;
#22483=CARTESIAN_POINT('Ctrl Pts',(-28.0118306429454,-6.92739322509109,
12.8579428468339)) ;
#22484=CARTESIAN_POINT('Ctrl Pts',(-26.9205390890661,-5.81959198653294,
9.28039690179885)) ;
#22485=CARTESIAN_POINT('Ctrl Pts',(-25.5975062439661,-4.49340440306587,
4.99035344644854)) ;
#22486=CARTESIAN_POINT('Ctrl Pts',(-24.696887404406,-3.61843630935476,2.13290843001981)) ;
#22487=CARTESIAN_POINT('Ctrl Pts',(-24.231863933635,-3.19121227129626,0.705454724400515)) ;
#22488=CARTESIAN_POINT('Ctrl Pts',(-23.9940039875064,-2.98789208895153,
-0.00956374451382109)) ;
#22489=CARTESIAN_POINT('Ctrl Pts',(-26.6659920777596,-7.59211093203314,
15.0017046656488)) ;
#22490=CARTESIAN_POINT('Ctrl Pts',(-26.2487210328116,-6.96393546602423,
12.8542436051414)) ;
#22491=CARTESIAN_POINT('Ctrl Pts',(-25.551936157679,-5.91719526611694,9.27528884741571)) ;
#22492=CARTESIAN_POINT('Ctrl Pts',(-24.7073383684488,-4.66179365816894,
4.9815562676005)) ;
#22493=CARTESIAN_POINT('Ctrl Pts',(-24.131376536521,-3.82821717034421,2.12007028295518)) ;
#22494=CARTESIAN_POINT('Ctrl Pts',(-23.8331919862405,-3.4144691374418,0.689960097960527)) ;
#22495=CARTESIAN_POINT('Ctrl Pts',(-23.6762514799622,-3.21253192150677,
-0.0250972881037275)) ;
#22496=CARTESIAN_POINT('Ctrl Pts',(-23.3332927479438,-7.5921558493803,14.9995815283504)) ;
#22497=CARTESIAN_POINT('Ctrl Pts',(-23.2961810253174,-6.98936415220679,
12.8516417322129)) ;
#22498=CARTESIAN_POINT('Ctrl Pts',(-23.2341794813628,-5.98449411694383,
9.27170531871678)) ;
#22499=CARTESIAN_POINT('Ctrl Pts',(-23.1590806809098,-4.7786211064264,4.975481034806)) ;
#22500=CARTESIAN_POINT('Ctrl Pts',(-23.1077088424374,-3.97369033142903,
2.11102719571202)) ;
#22501=CARTESIAN_POINT('Ctrl Pts',(-23.0810207228591,-3.57040548608313,
0.678584002796474)) ;
#22502=CARTESIAN_POINT('Ctrl Pts',(-23.0663319046393,-3.36714380447418,
-0.037695190406408)) ;
#22503=CARTESIAN_POINT('Ctrl Pts',(-20.0004784533517,-7.59212538979759,
15.0006756318296)) ;
#22504=CARTESIAN_POINT('Ctrl Pts',(-20.3389974659838,-6.97635407369755,
12.8529859672692)) ;
#22505=CARTESIAN_POINT('Ctrl Pts',(-20.904309853669,-5.95003859913919,9.27357788116746)) ;
#22506=CARTESIAN_POINT('Ctrl Pts',(-21.589449075084,-4.71871053547002,4.97864159456366)) ;
#22507=CARTESIAN_POINT('Ctrl Pts',(-22.0572141827788,-3.89911706770722,
2.11576153158121)) ;
#22508=CARTESIAN_POINT('Ctrl Pts',(-22.2997449599209,-3.49018725280383,
0.68467274594701)) ;
#22509=CARTESIAN_POINT('Ctrl Pts',(-22.4296586836676,-3.28819168978624,
-0.0306758267980919)) ;
#22510=CARTESIAN_POINT('Ctrl Pts',(-17.3345976129064,-7.59208088863895,
15.0047443273315)) ;
#22511=CARTESIAN_POINT('Ctrl Pts',(-17.9881563810077,-6.92728037248107,
12.8579470839996)) ;
#22512=CARTESIAN_POINT('Ctrl Pts',(-19.0794572594637,-5.81968155705656,
9.28034957582959)) ;
#22513=CARTESIAN_POINT('Ctrl Pts',(-20.4024577562282,-4.493316778673,4.99022917054663)) ;
#22514=CARTESIAN_POINT('Ctrl Pts',(-21.3030600185225,-3.61832290138349,
2.13278098397722)) ;
#22515=CARTESIAN_POINT('Ctrl Pts',(-21.7680877456986,-3.19093731667989,
0.705304501480531)) ;
#22516=CARTESIAN_POINT('Ctrl Pts',(-22.0059960124938,-2.98789208895172,
-0.00956374451383244)) ;
#22517=CARTESIAN_POINT('Ctrl Pts',(-16.0018526807048,-7.59210557221634,
15.0072731137197)) ;
#22518=CARTESIAN_POINT('Ctrl Pts',(-16.8207416298728,-6.896108115825,12.86098396712)) ;
#22519=CARTESIAN_POINT('Ctrl Pts',(-18.1877043400628,-5.73660744609285,
9.28448922209497)) ;
#22520=CARTESIAN_POINT('Ctrl Pts',(-19.8448445862136,-4.350203650837,4.99743947373445)) ;
#22521=CARTESIAN_POINT('Ctrl Pts',(-20.971600359406,-3.44029824352462,2.14308849921246)) ;
#22522=CARTESIAN_POINT('Ctrl Pts',(-21.5499907594839,-3.00195022998247,
0.716220735767196)) ;
#22523=CARTESIAN_POINT('Ctrl Pts',(-21.8410950678914,-2.79360243354798,
-5.70283445466835E-10)) ;
#22524=CARTESIAN_POINT('',(-16.2137002055612,-7.58988663107372,15.)) ;
#22525=CARTESIAN_POINT('Ctrl Pts',(-16.2137002055612,-7.58988663107372,
15.)) ;
#22526=CARTESIAN_POINT('Ctrl Pts',(-18.478683735487,-7.59137674406499,15.)) ;
#22527=CARTESIAN_POINT('Ctrl Pts',(-20.6776392287968,-7.59210830988921,
15.)) ;
#22528=CARTESIAN_POINT('Ctrl Pts',(-25.2082049599243,-7.59214580234589,
15.)) ;
#22529=CARTESIAN_POINT('Ctrl Pts',(-27.4623569795733,-7.59141553286644,
15.)) ;
#22530=CARTESIAN_POINT('Ctrl Pts',(-29.7862997944388,-7.58988663107372,
15.)) ;
#22531=CARTESIAN_POINT('',(-21.8072311118067,-2.82237333273713,0.089151802298673)) ;
#22532=CARTESIAN_POINT('Ctrl Pts',(-21.8072311118067,-2.82237333273713,
0.089151802298673)) ;
#22533=CARTESIAN_POINT('Ctrl Pts',(-21.8065429903626,-2.82295781693531,
0.0909648406217181)) ;
#22534=CARTESIAN_POINT('Ctrl Pts',(-21.8058548888846,-2.82354227570887,
0.0927779127895756)) ;
#22535=CARTESIAN_POINT('Ctrl Pts',(-21.8051668182352,-2.82412669991061,
0.0945909897307087)) ;
#22536=CARTESIAN_POINT('Ctrl Pts',(-21.3321463194345,-3.22589449435074,
1.34100741448435)) ;
#22537=CARTESIAN_POINT('Ctrl Pts',(-20.9412685773966,-3.55537108960553,
2.39676636675827)) ;
#22538=CARTESIAN_POINT('Ctrl Pts',(-19.998603574444,-4.35779260496273,4.91745775519203)) ;
#22539=CARTESIAN_POINT('Ctrl Pts',(-19.7551863923557,-4.56499578265944,
5.56835663524474)) ;
#22540=CARTESIAN_POINT('Ctrl Pts',(-19.4750304667258,-4.80369474586863,
6.31696808781126)) ;
#22541=CARTESIAN_POINT('Ctrl Pts',(-19.147214797811,-5.08330280289709,7.19178768834422)) ;
#22542=CARTESIAN_POINT('Ctrl Pts',(-19.0457931368179,-5.16980969155427,
7.4624448453042)) ;
#22543=CARTESIAN_POINT('Ctrl Pts',(-18.9398048742897,-5.2602370332511,7.74519133448698)) ;
#22544=CARTESIAN_POINT('Ctrl Pts',(-18.8343151585828,-5.35026227473964,
8.02651072809489)) ;
#22545=CARTESIAN_POINT('Ctrl Pts',(-17.9682804998251,-6.08933886405152,
10.3360471925039)) ;
#22546=CARTESIAN_POINT('Ctrl Pts',(-17.0532905544484,-6.87166393545832,
12.769529780144)) ;
#22547=CARTESIAN_POINT('Ctrl Pts',(-16.2137002055612,-7.58988663107372,
15.)) ;
#22548=CARTESIAN_POINT('',(-21.841095068034,-2.79360243342669,-4.72717753829954E-10)) ;
#22549=CARTESIAN_POINT('Ctrl Pts',(-21.84109506789,-2.79360243354897,-5.66911864674502E-10)) ;
#22550=CARTESIAN_POINT('Ctrl Pts',(-21.8304825380899,-2.8026212118579,0.0279159123264755)) ;
#22551=CARTESIAN_POINT('Ctrl Pts',(-21.8198816239617,-2.81162928529328,
0.0558291551528413)) ;
#22552=CARTESIAN_POINT('Ctrl Pts',(-21.8093004558439,-2.8206195620731,0.0837151694762296)) ;
#22553=CARTESIAN_POINT('Ctrl Pts',(-21.8086125788215,-2.82120401595886,
0.0855280268363439)) ;
#22554=CARTESIAN_POINT('Ctrl Pts',(-21.8079247354895,-2.82178843693437,
0.0873409002953505)) ;
#22555=CARTESIAN_POINT('Ctrl Pts',(-21.8072369214027,-2.82237282873864,
0.0891538007783507)) ;
#22556=CARTESIAN_POINT('Ctrl Pts',(-24.1589049323255,-2.79360243373209,
-2.99383723405346E-18)) ;
#22557=CARTESIAN_POINT('Ctrl Pts',(-24.041059962996,-2.93783796856924,-2.86693616357875E-18)) ;
#22558=CARTESIAN_POINT('Ctrl Pts',(-23.8975075094909,-3.05863551376881,
-1.87079518543243E-12)) ;
#22559=CARTESIAN_POINT('Ctrl Pts',(-23.5658814904478,-3.24512334221452,
-1.87079518543243E-12)) ;
#22560=CARTESIAN_POINT('Ctrl Pts',(-23.3797263777628,-3.30630896980136,
-6.13256942631573E-14)) ;
#22561=CARTESIAN_POINT('Ctrl Pts',(-22.9929117798555,-3.35479334786308,
-6.13261965942139E-14)) ;
#22562=CARTESIAN_POINT('Ctrl Pts',(-22.7955456606775,-3.34100668814767,
-1.18465996779747E-16)) ;
#22563=CARTESIAN_POINT('Ctrl Pts',(-22.453795578295,-3.24835176067042,-1.17553053613156E-16)) ;
#22564=CARTESIAN_POINT('Ctrl Pts',(-22.3085473875398,-3.18300649052949,
1.7646913418378E-13)) ;
#22565=CARTESIAN_POINT('Ctrl Pts',(-22.0497655129528,-3.01274318515093,
1.76470729940071E-13)) ;
#22566=CARTESIAN_POINT('Ctrl Pts',(-21.9368651572099,-2.91081957218221,
2.97818456042393E-17)) ;
#22567=CARTESIAN_POINT('Ctrl Pts',(-21.8410950676745,-2.79360243373208,
2.97352861784956E-17)) ;
#22568=CARTESIAN_POINT('Ctrl Pts',(-16.2120295002238,-7.79822359640593,
15.004760387006)) ;
#22569=CARTESIAN_POINT('Ctrl Pts',(-17.2939346788131,-6.86282814397786,
12.1445710778738)) ;
#22570=CARTESIAN_POINT('Ctrl Pts',(-18.916508261312,-5.45797832424605,7.85475085521625)) ;
#22571=CARTESIAN_POINT('Ctrl Pts',(-20.8015458475062,-3.79067453624556,
2.85615457147683)) ;
#22572=CARTESIAN_POINT('Ctrl Pts',(-21.5889562660143,-3.04704003130453,
0.715613732718789)) ;
#22573=CARTESIAN_POINT('Ctrl Pts',(-21.8410950678928,-2.79360243354618,
-5.74823466603647E-10)) ;
#22574=CARTESIAN_POINT('Ctrl Pts',(-16.2119914143525,-6.65586778828599,
15.0030622151785)) ;
#22575=CARTESIAN_POINT('Ctrl Pts',(-17.2645413499124,-5.90571197085084,
12.1423953161895)) ;
#22576=CARTESIAN_POINT('Ctrl Pts',(-18.8434539442202,-4.77886241298001,
7.85175076502351)) ;
#22577=CARTESIAN_POINT('Ctrl Pts',(-20.6801468481248,-3.44148597527413,
2.8497432463707)) ;
#22578=CARTESIAN_POINT('Ctrl Pts',(-21.4549018244985,-2.84279904912998,
0.707828841050375)) ;
#22579=CARTESIAN_POINT('Ctrl Pts',(-21.7046665053844,-2.63588685245852,
-0.00706604194226517)) ;
#22580=CARTESIAN_POINT('Ctrl Pts',(-16.2119015637445,-4.37088429774524,
15.0004367897856)) ;
#22581=CARTESIAN_POINT('Ctrl Pts',(-17.2199451957636,-3.97936993493365,
12.1389905639006)) ;
#22582=CARTESIAN_POINT('Ctrl Pts',(-18.7323433798125,-3.39144877186261,
7.8469202359414)) ;
#22583=CARTESIAN_POINT('Ctrl Pts',(-20.4957476119421,-2.6929916740198,2.83991086222072)) ;
#22584=CARTESIAN_POINT('Ctrl Pts',(-21.2501213955004,-2.37937043746566,
0.694489603884554)) ;
#22585=CARTESIAN_POINT('Ctrl Pts',(-21.4999730616134,-2.2671878990079,-0.0206641948568487)) ;
#22586=CARTESIAN_POINT('Ctrl Pts',(-16.2118565250724,-0.371717894292294,
14.9994437267388)) ;
#22587=CARTESIAN_POINT('Ctrl Pts',(-17.2034970653009,-0.588656421028745,
12.1376935596273)) ;
#22588=CARTESIAN_POINT('Ctrl Pts',(-18.6908746045858,-0.914396456191195,
7.84496467022684)) ;
#22589=CARTESIAN_POINT('Ctrl Pts',(-20.4272574580087,-1.3014899842262,2.83611936781098)) ;
#22590=CARTESIAN_POINT('Ctrl Pts',(-21.173694786691,-1.47529391663119,0.688887749999729)) ;
#22591=CARTESIAN_POINT('Ctrl Pts',(-21.4246891608723,-1.53804477792109,
-0.0267691804533001)) ;
#22592=CARTESIAN_POINT('Ctrl Pts',(-16.2119723714168,2.4846898842279,15.0022131292648)) ;
#22593=CARTESIAN_POINT('Ctrl Pts',(-17.2497059688142,1.82724833732013,12.1413021811523)) ;
#22594=CARTESIAN_POINT('Ctrl Pts',(-18.8070103620793,0.839346881044636,
7.85030531659959)) ;
#22595=CARTESIAN_POINT('Ctrl Pts',(-20.6193140212913,-0.332972447041589,
2.84662301371282)) ;
#22596=CARTESIAN_POINT('Ctrl Pts',(-21.3876763824965,-0.85887468237252,
0.70401123140127)) ;
#22597=CARTESIAN_POINT('Ctrl Pts',(-21.6364522241304,-1.04297093808501,
-0.0105990626259748)) ;
#22598=CARTESIAN_POINT('Ctrl Pts',(-16.2120295002238,4.19822359640781,15.004760387006)) ;
#22599=CARTESIAN_POINT('Ctrl Pts',(-17.2939346788131,3.26282814397944,12.1445710778738)) ;
#22600=CARTESIAN_POINT('Ctrl Pts',(-18.9165082613121,1.85797832424717,7.85475085521625)) ;
#22601=CARTESIAN_POINT('Ctrl Pts',(-20.8015458475064,0.190674536246134,
2.85615457147684)) ;
#22602=CARTESIAN_POINT('Ctrl Pts',(-21.5889562660145,-0.552959968695133,
0.715613732718802)) ;
#22603=CARTESIAN_POINT('Ctrl Pts',(-21.8410950678931,-0.806397566453563,
-5.74811837017464E-10)) ;
#22604=CARTESIAN_POINT('',(-16.2137002055612,3.98988663107372,15.)) ;
#22605=CARTESIAN_POINT('Ctrl Pts',(-16.2137002055612,3.98988663107372,15.)) ;
#22606=CARTESIAN_POINT('Ctrl Pts',(-16.2125145547255,2.07140621568792,15.)) ;
#22607=CARTESIAN_POINT('Ctrl Pts',(-16.2119115973002,0.183463303037694,
15.)) ;
#22608=CARTESIAN_POINT('Ctrl Pts',(-16.2118809961308,-3.68622209538906,
15.)) ;
#22609=CARTESIAN_POINT('Ctrl Pts',(-16.2124839012804,-5.62180642421694,
15.)) ;
#22610=CARTESIAN_POINT('Ctrl Pts',(-16.2137002055612,-7.58988663107371,
15.)) ;
#22611=CARTESIAN_POINT('',(-21.8072311118067,-0.77762666726287,0.089151802298673)) ;
#22612=CARTESIAN_POINT('Ctrl Pts',(-21.8072311118067,-0.77762666726287,
0.089151802298673)) ;
#22613=CARTESIAN_POINT('Ctrl Pts',(-21.8065429885505,-0.777042181525532,
0.0909648453961011)) ;
#22614=CARTESIAN_POINT('Ctrl Pts',(-21.805854890698,-0.776457725828476,
0.0927779080151138)) ;
#22615=CARTESIAN_POINT('Ctrl Pts',(-21.8051668182363,-0.775873300088152,
0.0945909897307308)) ;
#22616=CARTESIAN_POINT('Ctrl Pts',(-21.3321456286191,-0.374104918924787,
1.34100923475312)) ;
#22617=CARTESIAN_POINT('Ctrl Pts',(-20.9412686792828,-0.0446289960646136,
2.3967660917748)) ;
#22618=CARTESIAN_POINT('Ctrl Pts',(-19.9986040235856,0.757792222641507,
4.91745655418507)) ;
#22619=CARTESIAN_POINT('Ctrl Pts',(-19.7551865550768,0.964995643873722,
5.5683562007834)) ;
#22620=CARTESIAN_POINT('Ctrl Pts',(-19.4750302004634,1.20369497249373,6.31696880020665)) ;
#22621=CARTESIAN_POINT('Ctrl Pts',(-19.1472138763084,1.48330358888621,7.19179014749615)) ;
#22622=CARTESIAN_POINT('Ctrl Pts',(-19.0457924000719,1.5698103201055,7.46244681083961)) ;
#22623=CARTESIAN_POINT('Ctrl Pts',(-18.9398043540903,1.66023747714745,7.74519272193313)) ;
#22624=CARTESIAN_POINT('Ctrl Pts',(-18.8343148546405,1.75026253412495,8.02651153864665)) ;
#22625=CARTESIAN_POINT('Ctrl Pts',(-17.9682802857615,2.48933904709054,10.3360477618804)) ;
#22626=CARTESIAN_POINT('Ctrl Pts',(-17.0532904562273,3.27166401948096,12.7695300410798)) ;
#22627=CARTESIAN_POINT('Ctrl Pts',(-16.2137002055612,3.98988663107372,15.)) ;
#22628=CARTESIAN_POINT('',(-21.841095068039,-0.806397566577556,-4.79304988060258E-10)) ;
#22629=CARTESIAN_POINT('Ctrl Pts',(-21.841095067893,-0.806397566453594,
-5.74813162346199E-10)) ;
#22630=CARTESIAN_POINT('Ctrl Pts',(-21.8304825311591,-0.797378782252167,
0.0279159305576807)) ;
#22631=CARTESIAN_POINT('Ctrl Pts',(-21.8198806143693,-0.788372087620017,
0.0558294110268321)) ;
#22632=CARTESIAN_POINT('Ctrl Pts',(-21.8092977142497,-0.779384122982931,
0.0837157785108199)) ;
#22633=CARTESIAN_POINT('Ctrl Pts',(-21.8086097266589,-0.778799821131193,
0.0855286534849715)) ;
#22634=CARTESIAN_POINT('Ctrl Pts',(-21.8079217617944,-0.778215549506057,
0.0873415657621646)) ;
#22635=CARTESIAN_POINT('Ctrl Pts',(-21.8072338308928,-0.777631317536321,
0.0891544850728279)) ;
#22636=CARTESIAN_POINT('Ctrl Pts',(-21.8410950676745,-2.79360243373211,
1.7888651467981E-16)) ;
#22637=CARTESIAN_POINT('Ctrl Pts',(-21.716402375793,-2.6542834674913,1.78818550473223E-16)) ;
#22638=CARTESIAN_POINT('Ctrl Pts',(-21.6191945405804,-2.49286283644828,
-1.18389961251751E-12)) ;
#22639=CARTESIAN_POINT('Ctrl Pts',(-21.487197585082,-2.13565023378541,-1.1839008088782E-12)) ;
#22640=CARTESIAN_POINT('Ctrl Pts',(-21.4561344460552,-1.94241064629152,
-1.40165656858926E-15)) ;
#22641=CARTESIAN_POINT('Ctrl Pts',(-21.4688023848785,-1.57296219574121,
-1.40165656858926E-15)) ;
#22642=CARTESIAN_POINT('Ctrl Pts',(-21.5058130688892,-1.39951177553656,
1.45716771982052E-14)) ;
#22643=CARTESIAN_POINT('Ctrl Pts',(-21.6365692781991,-1.07876898953231,
1.45716771982052E-14)) ;
#22644=CARTESIAN_POINT('Ctrl Pts',(-21.7274655448062,-0.933355669598461,
-1.29039860188898E-16)) ;
#22645=CARTESIAN_POINT('Ctrl Pts',(-21.8410950676745,-0.806397566267894,
-1.29036351619964E-16)) ;
#22646=CARTESIAN_POINT('Ctrl Pts',(-16.001852680703,3.99210557221634,15.0072731137197)) ;
#22647=CARTESIAN_POINT('Ctrl Pts',(-16.8207416298715,3.29610811582475,12.8609839671193)) ;
#22648=CARTESIAN_POINT('Ctrl Pts',(-18.1877024573399,2.13660628597323,9.28448888442423)) ;
#22649=CARTESIAN_POINT('Ctrl Pts',(-19.844842964605,0.750203431437901,4.99743893001117)) ;
#22650=CARTESIAN_POINT('Ctrl Pts',(-20.9715983994063,-0.159702216928202,
2.14308790534903)) ;
#22651=CARTESIAN_POINT('Ctrl Pts',(-21.5499907594854,-0.598049770019083,
0.716220735762898)) ;
#22652=CARTESIAN_POINT('Ctrl Pts',(-21.841095067893,-0.806397566453593,
-5.74812294984461E-10)) ;
#22653=CARTESIAN_POINT('Ctrl Pts',(-16.6682251468039,3.99209323042764,15.0060087205256)) ;
#22654=CARTESIAN_POINT('Ctrl Pts',(-17.4045039137444,3.31167027710832,12.8594663783478)) ;
#22655=CARTESIAN_POINT('Ctrl Pts',(-18.6335549140447,2.17813825733505,9.28242868527079)) ;
#22656=CARTESIAN_POINT('Ctrl Pts',(-20.1237719122027,0.821772347358335,
4.99388557690666)) ;
#22657=CARTESIAN_POINT('Ctrl Pts',(-21.1374684967843,-0.0707256802637752,
2.13799104359245)) ;
#22658=CARTESIAN_POINT('Ctrl Pts',(-21.6593105354534,-0.503423080828448,
0.710881903949976)) ;
#22659=CARTESIAN_POINT('Ctrl Pts',(-21.9235455401941,-0.709252738751684,
-0.00478187254658313)) ;
#22660=CARTESIAN_POINT('Ctrl Pts',(-18.6674857660828,3.99209091164725,15.0025729768987)) ;
#22661=CARTESIAN_POINT('Ctrl Pts',(-19.1614746123909,3.35363082901585,12.855308289841)) ;
#22662=CARTESIAN_POINT('Ctrl Pts',(-19.9863755029411,2.28972627060116,9.2767748169095)) ;
#22663=CARTESIAN_POINT('Ctrl Pts',(-20.9863676148636,1.01425473330893,4.98409359929946)) ;
#22664=CARTESIAN_POINT('Ctrl Pts',(-21.6680397534922,0.168983505203374,
2.12382823604792)) ;
#22665=CARTESIAN_POINT('Ctrl Pts',(-22.0210644484083,-0.248866124683977,
0.694779644890225)) ;
#22666=CARTESIAN_POINT('Ctrl Pts',(-22.2056967668507,-0.450222874926842,
-0.0198469372912451)) ;
#22667=CARTESIAN_POINT('Ctrl Pts',(-22.0001427064207,3.99216271493084,14.9993531978443)) ;
#22668=CARTESIAN_POINT('Ctrl Pts',(-22.1123412771431,3.39200499629872,12.8513619624513)) ;
#22669=CARTESIAN_POINT('Ctrl Pts',(-22.2996679554014,2.39168358729901,9.2712991683703)) ;
#22670=CARTESIAN_POINT('Ctrl Pts',(-22.5266934010037,1.19099399650789,4.97478325695134)) ;
#22671=CARTESIAN_POINT('Ctrl Pts',(-22.6818522659833,0.389104720411302,
2.1100005997556)) ;
#22672=CARTESIAN_POINT('Ctrl Pts',(-22.7622868668625,-0.013113282879768,
0.677230000874634)) ;
#22673=CARTESIAN_POINT('Ctrl Pts',(-22.806110018343,-0.216603976952604,
-0.0391821457269935)) ;
#22674=CARTESIAN_POINT('Ctrl Pts',(-25.9995219192719,3.99212515591032,15.0006787361289)) ;
#22675=CARTESIAN_POINT('Ctrl Pts',(-25.6610300798093,3.37631293153872,12.85299059408)) ;
#22676=CARTESIAN_POINT('Ctrl Pts',(-25.0957200971754,2.34995910229997,9.27358133907209)) ;
#22677=CARTESIAN_POINT('Ctrl Pts',(-24.4106656326799,1.11857404454784,4.97865384323633)) ;
#22678=CARTESIAN_POINT('Ctrl Pts',(-23.9429141916785,0.298927109368283,
2.11577890293457)) ;
#22679=CARTESIAN_POINT('Ctrl Pts',(-23.7004725142412,-0.109962398029831,
0.684723933467854)) ;
#22680=CARTESIAN_POINT('Ctrl Pts',(-23.5704121779659,-0.311946932728745,
-0.030647716704717)) ;
#22681=CARTESIAN_POINT('Ctrl Pts',(-28.6654023870944,3.99208088863895,15.0047443273315)) ;
#22682=CARTESIAN_POINT('Ctrl Pts',(-28.0118267664842,3.32730856489621,12.8579460343649)) ;
#22683=CARTESIAN_POINT('Ctrl Pts',(-26.9205516217294,2.21967036822145,9.28035754568041)) ;
#22684=CARTESIAN_POINT('Ctrl Pts',(-25.5975051802046,0.893334293744912,
4.99023689930695)) ;
#22685=CARTESIAN_POINT('Ctrl Pts',(-24.6969016254348,0.0183616639676227,
2.13278867184277)) ;
#22686=CARTESIAN_POINT('Ctrl Pts',(-24.2318215462195,-0.409050652094805,
0.705292734981902)) ;
#22687=CARTESIAN_POINT('Ctrl Pts',(-23.9940039875048,-0.61210791104966,
-0.00956374451836098)) ;
#22688=CARTESIAN_POINT('Ctrl Pts',(-29.9981473192961,3.99210557221634,15.0072731137197)) ;
#22689=CARTESIAN_POINT('Ctrl Pts',(-29.1792583701277,3.29610811582477,12.8609839671193)) ;
#22690=CARTESIAN_POINT('Ctrl Pts',(-27.8122975426595,2.13660628597329,9.28448888442423)) ;
#22691=CARTESIAN_POINT('Ctrl Pts',(-26.1551570353946,0.750203431438,4.99743893001117)) ;
#22692=CARTESIAN_POINT('Ctrl Pts',(-25.0284016005935,-0.159702216928078,
2.14308790534903)) ;
#22693=CARTESIAN_POINT('Ctrl Pts',(-24.4500092405145,-0.598049770018951,
0.71622073576289)) ;
#22694=CARTESIAN_POINT('Ctrl Pts',(-24.1589049321068,-0.806397566453458,
-5.74818942444821E-10)) ;
#22695=CARTESIAN_POINT('Ctrl Pts',(-29.7862997944388,3.98988663107372,15.)) ;
#22696=CARTESIAN_POINT('Ctrl Pts',(-27.5213162645095,3.99137674406499,15.)) ;
#22697=CARTESIAN_POINT('Ctrl Pts',(-25.3223607712015,3.99210830988921,15.)) ;
#22698=CARTESIAN_POINT('Ctrl Pts',(-20.7917950400773,3.99214580234589,15.)) ;
#22699=CARTESIAN_POINT('Ctrl Pts',(-18.5376430204301,3.99141553286645,15.)) ;
#22700=CARTESIAN_POINT('Ctrl Pts',(-16.2137002055612,3.98988663107372,15.)) ;
#22701=CARTESIAN_POINT('Ctrl Pts',(-21.8410950676745,-0.806397566267961,
2.12829438470106E-16)) ;
#22702=CARTESIAN_POINT('Ctrl Pts',(-21.9589400370039,-0.66216203143079,
2.11480923218598E-16)) ;
#22703=CARTESIAN_POINT('Ctrl Pts',(-22.1024924905091,-0.541364486231195,
-1.87079518543243E-12)) ;
#22704=CARTESIAN_POINT('Ctrl Pts',(-22.4341185095522,-0.354876657785478,
-1.87079518543243E-12)) ;
#22705=CARTESIAN_POINT('Ctrl Pts',(-22.6202736222372,-0.29369103019864,
-6.13118164753495E-14)) ;
#22706=CARTESIAN_POINT('Ctrl Pts',(-23.0070882201445,-0.245206652136923,
-6.13123188064061E-14)) ;
#22707=CARTESIAN_POINT('Ctrl Pts',(-23.2044543393225,-0.258993311852331,
-1.53160466299283E-16)) ;
#22708=CARTESIAN_POINT('Ctrl Pts',(-23.546204421705,-0.35164823932958,-1.52247523132693E-16)) ;
#22709=CARTESIAN_POINT('Ctrl Pts',(-23.6914526124602,-0.416993509470512,
1.76455256395972E-13)) ;
#22710=CARTESIAN_POINT('Ctrl Pts',(-23.9502344870472,-0.587256814849067,
1.76456852152263E-13)) ;
#22711=CARTESIAN_POINT('Ctrl Pts',(-24.0631348427901,-0.689180427817769,
6.92945052858629E-17)) ;
#22712=CARTESIAN_POINT('Ctrl Pts',(-24.1589049323255,-0.806397566267902,
6.93843681060263E-17)) ;
#22713=CARTESIAN_POINT('Origin',(-23.,-1.8,0.)) ;
#22714=CARTESIAN_POINT('',(-24.3286990541393,-0.661115096452054,0.)) ;
#22715=CARTESIAN_POINT('',(-24.3286990541393,-2.93888490354795,0.)) ;
#22716=CARTESIAN_POINT('Origin',(-23.,-1.8,0.)) ;
#22717=CARTESIAN_POINT('',(-21.6713009458607,-0.661115096452054,0.)) ;
#22718=CARTESIAN_POINT('Origin',(-23.,-1.8,0.)) ;
#22719=CARTESIAN_POINT('',(-21.6713009458607,-2.93888490354795,0.)) ;
#22720=CARTESIAN_POINT('Origin',(-23.,-1.8,0.)) ;
#22721=CARTESIAN_POINT('Origin',(-23.,-1.8,0.)) ;
#22722=CARTESIAN_POINT('Origin',(-23.,-1.8,15.)) ;
#22723=CARTESIAN_POINT('',(-30.,4.2,15.)) ;
#22724=CARTESIAN_POINT('',(-30.,-7.8,15.)) ;
#22725=CARTESIAN_POINT('',(-30.,4.2,15.)) ;
#22726=CARTESIAN_POINT('',(-16.,-7.8,15.)) ;
#22727=CARTESIAN_POINT('',(-30.,-7.8,15.)) ;
#22728=CARTESIAN_POINT('',(-16.,4.2,15.)) ;
#22729=CARTESIAN_POINT('',(-16.,-7.8,15.)) ;
#22730=CARTESIAN_POINT('',(-16.,4.2,15.)) ;
#22731=CARTESIAN_POINT('Ctrl Pts',(-30.,4.2,15.)) ;
#22732=CARTESIAN_POINT('Ctrl Pts',(-28.1095663513798,2.57962830118265,10.)) ;
#22733=CARTESIAN_POINT('Ctrl Pts',(-26.2191327027595,0.959256602365297,
5.)) ;
#22734=CARTESIAN_POINT('Ctrl Pts',(-24.3286990541393,-0.661115096452054,
0.)) ;
#22735=CARTESIAN_POINT('Ctrl Pts',(-30.,3.05714285714286,15.)) ;
#22736=CARTESIAN_POINT('Ctrl Pts',(-28.1608824747724,1.75795796494175,9.99999999999999)) ;
#22737=CARTESIAN_POINT('Ctrl Pts',(-26.3215392010018,0.458726737174903,
5.00000000000001)) ;
#22738=CARTESIAN_POINT('Ctrl Pts',(-24.4824216757743,-0.840458155026201,
0.)) ;
#22739=CARTESIAN_POINT('Ctrl Pts',(-30.,0.77142857142857,15.)) ;
#22740=CARTESIAN_POINT('Ctrl Pts',(-28.2386698968374,0.0935987464520723,
10.)) ;
#22741=CARTESIAN_POINT('Ctrl Pts',(-26.4768558425974,-0.584062875210304,
4.99999999999999)) ;
#22742=CARTESIAN_POINT('Ctrl Pts',(-24.7155257394348,-1.2618927001868,0.)) ;
#22743=CARTESIAN_POINT('Ctrl Pts',(-30.,-3.22857142857143,15.)) ;
#22744=CARTESIAN_POINT('Ctrl Pts',(-28.2673008175541,-2.85300906076429,
9.99999999999999)) ;
#22745=CARTESIAN_POINT('Ctrl Pts',(-26.5346802019186,-2.47747049404618,
5.00000000000001)) ;
#22746=CARTESIAN_POINT('Ctrl Pts',(-24.8019810194727,-2.10190812623904,
0.)) ;
#22747=CARTESIAN_POINT('Ctrl Pts',(-30.,-6.08571428571429,15.)) ;
#22748=CARTESIAN_POINT('Ctrl Pts',(-28.1867947927088,-4.94728771311918,
10.)) ;
#22749=CARTESIAN_POINT('Ctrl Pts',(-26.372488193883,-3.80829688828183,5.)) ;
#22750=CARTESIAN_POINT('Ctrl Pts',(-24.5592829865917,-2.66987031568673,
0.)) ;
#22751=CARTESIAN_POINT('Ctrl Pts',(-30.,-7.8,15.)) ;
#22752=CARTESIAN_POINT('Ctrl Pts',(-28.1095663513798,-6.17962830118265,
10.)) ;
#22753=CARTESIAN_POINT('Ctrl Pts',(-26.2191327027595,-4.5592566023653,5.)) ;
#22754=CARTESIAN_POINT('Ctrl Pts',(-24.3286990541393,-2.93888490354795,
0.)) ;
#22755=CARTESIAN_POINT('',(-30.,4.2,15.)) ;
#22756=CARTESIAN_POINT('',(-30.,-7.8,15.)) ;
#22757=CARTESIAN_POINT('Ctrl Pts',(-30.,-7.8,15.)) ;
#22758=CARTESIAN_POINT('Ctrl Pts',(-28.1095663513798,-6.17962830118265,
10.)) ;
#22759=CARTESIAN_POINT('Ctrl Pts',(-26.2191327027595,-4.5592566023653,5.)) ;
#22760=CARTESIAN_POINT('Ctrl Pts',(-24.3286990541393,-2.93888490354795,
0.)) ;
#22761=CARTESIAN_POINT('Ctrl Pts',(-28.6666666666667,-7.8,15.)) ;
#22762=CARTESIAN_POINT('Ctrl Pts',(-27.1584336023967,-6.25242905179828,
10.)) ;
#22763=CARTESIAN_POINT('Ctrl Pts',(-25.6499011737328,-4.70465862053891,
5.)) ;
#22764=CARTESIAN_POINT('Ctrl Pts',(-24.1416681094628,-3.15708767233719,
0.)) ;
#22765=CARTESIAN_POINT('Ctrl Pts',(-26.,-7.8,15.)) ;
#22766=CARTESIAN_POINT('Ctrl Pts',(-25.2193650979419,-6.36643657871293,
10.)) ;
#22767=CARTESIAN_POINT('Ctrl Pts',(-24.4387564842615,-4.93275627338872,
5.00000000000001)) ;
#22768=CARTESIAN_POINT('Ctrl Pts',(-23.6581215822033,-3.49919285210164,
0.)) ;
#22769=CARTESIAN_POINT('Ctrl Pts',(-22.,-7.8,15.)) ;
#22770=CARTESIAN_POINT('Ctrl Pts',(-22.2587099775723,-6.40287188477929,
10.)) ;
#22771=CARTESIAN_POINT('Ctrl Pts',(-22.5172538720266,-5.00574529287019,
4.99999999999999)) ;
#22772=CARTESIAN_POINT('Ctrl Pts',(-22.7759638495989,-3.60861717764948,
0.)) ;
#22773=CARTESIAN_POINT('Ctrl Pts',(-18.6666666666667,-7.8,15.)) ;
#22774=CARTESIAN_POINT('Ctrl Pts',(-19.8062578158211,-6.31371238783143,
10.)) ;
#22775=CARTESIAN_POINT('Ctrl Pts',(-20.9459555636257,-4.82732800860068,
5.)) ;
#22776=CARTESIAN_POINT('Ctrl Pts',(-22.0855467127802,-3.34104039643211,
0.)) ;
#22777=CARTESIAN_POINT('Ctrl Pts',(-16.6666666666667,-7.8,15.)) ;
#22778=CARTESIAN_POINT('Ctrl Pts',(-18.3661025308913,-6.21593369039753,
10.)) ;
#22779=CARTESIAN_POINT('Ctrl Pts',(-20.0653805539744,-4.63205259754504,
5.)) ;
#22780=CARTESIAN_POINT('Ctrl Pts',(-21.764816418199,-3.04798628794257,0.)) ;
#22781=CARTESIAN_POINT('Ctrl Pts',(-16.,-7.8,15.)) ;
#22782=CARTESIAN_POINT('Ctrl Pts',(-17.8904336486202,-6.17962830118265,
10.)) ;
#22783=CARTESIAN_POINT('Ctrl Pts',(-19.7808672972405,-4.5592566023653,5.)) ;
#22784=CARTESIAN_POINT('Ctrl Pts',(-21.6713009458607,-2.93888490354795,
0.)) ;
#22785=CARTESIAN_POINT('',(-16.,-7.8,15.)) ;
#22786=CARTESIAN_POINT('Ctrl Pts',(-16.,-7.8,15.)) ;
#22787=CARTESIAN_POINT('Ctrl Pts',(-17.8904336486202,-6.17962830118265,
10.)) ;
#22788=CARTESIAN_POINT('Ctrl Pts',(-19.7808672972405,-4.5592566023653,5.)) ;
#22789=CARTESIAN_POINT('Ctrl Pts',(-21.6713009458607,-2.93888490354795,
0.)) ;
#22790=CARTESIAN_POINT('Ctrl Pts',(-16.,-6.65714285714286,15.)) ;
#22791=CARTESIAN_POINT('Ctrl Pts',(-17.8391086044718,-5.35795456184796,
10.)) ;
#22792=CARTESIAN_POINT('Ctrl Pts',(-19.678469719754,-4.0587301402687,4.99999999999999)) ;
#22793=CARTESIAN_POINT('Ctrl Pts',(-21.5175783242257,-2.7595418449738,0.)) ;
#22794=CARTESIAN_POINT('Ctrl Pts',(-16.,-4.37142857142857,15.)) ;
#22795=CARTESIAN_POINT('Ctrl Pts',(-17.7613419010902,-3.69360594086809,
9.99999999999998)) ;
#22796=CARTESIAN_POINT('Ctrl Pts',(-19.5231801272942,-3.01597519408864,
5.00000000000002)) ;
#22797=CARTESIAN_POINT('Ctrl Pts',(-21.2845220283845,-2.33815256352815,
0.)) ;
#22798=CARTESIAN_POINT('Ctrl Pts',(-16.,-0.371428571428572,15.)) ;
#22799=CARTESIAN_POINT('Ctrl Pts',(-17.732695160094,-0.746986389367562,
10.)) ;
#22800=CARTESIAN_POINT('Ctrl Pts',(-19.4652823817506,-1.12245808880451,
4.99999999999999)) ;
#22801=CARTESIAN_POINT('Ctrl Pts',(-21.1979775418446,-1.4980159067435,0.)) ;
#22802=CARTESIAN_POINT('Ctrl Pts',(-16.,2.48571428571428,15.)) ;
#22803=CARTESIAN_POINT('Ctrl Pts',(-17.8132062724847,1.34728533115534,9.99999999999999)) ;
#22804=CARTESIAN_POINT('Ctrl Pts',(-19.6275107409235,0.208299270245674,
5.00000000000001)) ;
#22805=CARTESIAN_POINT('Ctrl Pts',(-21.4407170134083,-0.930129684313275,
0.)) ;
#22806=CARTESIAN_POINT('Ctrl Pts',(-16.,4.2,15.)) ;
#22807=CARTESIAN_POINT('Ctrl Pts',(-17.8904336486202,2.57962830118265,10.)) ;
#22808=CARTESIAN_POINT('Ctrl Pts',(-19.7808672972405,0.959256602365297,
5.)) ;
#22809=CARTESIAN_POINT('Ctrl Pts',(-21.6713009458607,-0.661115096452054,
0.)) ;
#22810=CARTESIAN_POINT('',(-16.,4.2,15.)) ;
#22811=CARTESIAN_POINT('Ctrl Pts',(-16.,4.2,15.)) ;
#22812=CARTESIAN_POINT('Ctrl Pts',(-17.8904336486202,2.57962830118265,10.)) ;
#22813=CARTESIAN_POINT('Ctrl Pts',(-19.7808672972405,0.959256602365298,
5.)) ;
#22814=CARTESIAN_POINT('Ctrl Pts',(-21.6713009458607,-0.661115096452054,
0.)) ;
#22815=CARTESIAN_POINT('Ctrl Pts',(-17.3333333333333,4.2,15.)) ;
#22816=CARTESIAN_POINT('Ctrl Pts',(-18.8415663976033,2.65242905179828,10.)) ;
#22817=CARTESIAN_POINT('Ctrl Pts',(-20.3500988262672,1.10465862053891,5.)) ;
#22818=CARTESIAN_POINT('Ctrl Pts',(-21.8583318905372,-0.442912327662807,
0.)) ;
#22819=CARTESIAN_POINT('Ctrl Pts',(-20.,4.2,15.)) ;
#22820=CARTESIAN_POINT('Ctrl Pts',(-20.7806349020582,2.76643657871293,9.99999999999999)) ;
#22821=CARTESIAN_POINT('Ctrl Pts',(-21.5612412315327,1.33275849418373,5.00000000000001)) ;
#22822=CARTESIAN_POINT('Ctrl Pts',(-22.3418761335909,-0.100804927103342,
0.)) ;
#22823=CARTESIAN_POINT('Ctrl Pts',(-24.,4.2,15.)) ;
#22824=CARTESIAN_POINT('Ctrl Pts',(-23.7412900224277,2.80287188477929,10.)) ;
#22825=CARTESIAN_POINT('Ctrl Pts',(-23.4827448088328,1.40574635303797,4.99999999999999)) ;
#22826=CARTESIAN_POINT('Ctrl Pts',(-23.2240348312605,0.00861823781726209,
0.)) ;
#22827=CARTESIAN_POINT('Ctrl Pts',(-27.3333333333333,4.2,15.)) ;
#22828=CARTESIAN_POINT('Ctrl Pts',(-26.1937421841789,2.71371238783143,10.)) ;
#22829=CARTESIAN_POINT('Ctrl Pts',(-25.054043528944,1.22732858634997,5.)) ;
#22830=CARTESIAN_POINT('Ctrl Pts',(-23.9144523797896,-0.258959025818595,
0.)) ;
#22831=CARTESIAN_POINT('Ctrl Pts',(-29.3333333333333,4.2,15.)) ;
#22832=CARTESIAN_POINT('Ctrl Pts',(-27.6338974691087,2.61593369039753,10.)) ;
#22833=CARTESIAN_POINT('Ctrl Pts',(-25.9346194460256,1.03205259754504,5.)) ;
#22834=CARTESIAN_POINT('Ctrl Pts',(-24.235183581801,-0.55201371205743,0.)) ;
#22835=CARTESIAN_POINT('Ctrl Pts',(-30.,4.2,15.)) ;
#22836=CARTESIAN_POINT('Ctrl Pts',(-28.1095663513798,2.57962830118265,10.)) ;
#22837=CARTESIAN_POINT('Ctrl Pts',(-26.2191327027595,0.959256602365298,
5.)) ;
#22838=CARTESIAN_POINT('Ctrl Pts',(-24.3286990541393,-0.661115096452054,
0.)) ;
#24555=UNCERTAINTY_MEASURE_WITH_UNIT(LENGTH_MEASURE(0.001),#24629,
'DISTANCE_ACCURACY_VALUE',
'Maximum model space distance between geometric entities at asserted c
onnectivities') ;
#24580=UNCERTAINTY_MEASURE_WITH_UNIT(LENGTH_MEASURE(0.001),#24629,
'DISTANCE_ACCURACY_VALUE',
'Maximum model space distance between geometric entities at asserted c
onnectivities') ;
#24603=(
GEOMETRIC_REPRESENTATION_CONTEXT(3)
GLOBAL_UNCERTAINTY_ASSIGNED_CONTEXT((#24555))
GLOBAL_UNIT_ASSIGNED_CONTEXT((#24629,#24631,#24632))
REPRESENTATION_CONTEXT('','3D')
) ;
#24628=(
GEOMETRIC_REPRESENTATION_CONTEXT(3)
GLOBAL_UNCERTAINTY_ASSIGNED_CONTEXT((#24580))
GLOBAL_UNIT_ASSIGNED_CONTEXT((#24629,#24631,#24632))
REPRESENTATION_CONTEXT('','3D')
) ;
#24629=(
LENGTH_UNIT()
NAMED_UNIT(*)
SI_UNIT(.CENTI.,.METRE.)
) ;
#24631=(
NAMED_UNIT(*)
PLANE_ANGLE_UNIT()
SI_UNIT($,.RADIAN.)
) ;
#24632=(
NAMED_UNIT(*)
SI_UNIT($,.STERADIAN.)
SOLID_ANGLE_UNIT()
) ;
#24655=SHAPE_DEFINITION_REPRESENTATION(#24724,#24813) ;
#24724=PRODUCT_DEFINITION_SHAPE('',$,#24861) ;
#24813=SHAPE_REPRESENTATION('',(#14856),#24603) ;
#24838=PRODUCT_DEFINITION_CONTEXT('part definition',#24981,'design') ;
#24861=PRODUCT_DEFINITION('SEED_FEED_HOPPER','SEED_FEED_HOPPER',
#24908,#24838) ;
#24908=PRODUCT_DEFINITION_FORMATION('',$,#25005) ;
#24981=APPLICATION_CONTEXT(
'Core Data for Automotive Mechanical Design Process') ;
#24982=PRODUCT_CONTEXT('part definition',#24981,'mechanical') ;
#25005=PRODUCT('SEED_FEED_HOPPER','SEED_FEED_HOPPER',$,(#24982)) ;
#25038=PRESENTATION_STYLE_ASSIGNMENT((#25048)) ;
#25048=SURFACE_STYLE_USAGE(.BOTH.,#25058) ;
#25058=SURFACE_SIDE_STYLE('',(#25068)) ;
#25068=SURFACE_STYLE_FILL_AREA(#25078) ;
#25078=FILL_AREA_STYLE('Surface - Matte',(#25088)) ;
#25088=FILL_AREA_STYLE_COLOUR('Surface - Matte',#25098) ;
#25098=COLOUR_RGB('Surface - Matte', 0.66274510, 0.83137255, 0.94901961) ;
ENDSEC;
END-ISO-10303-21;
